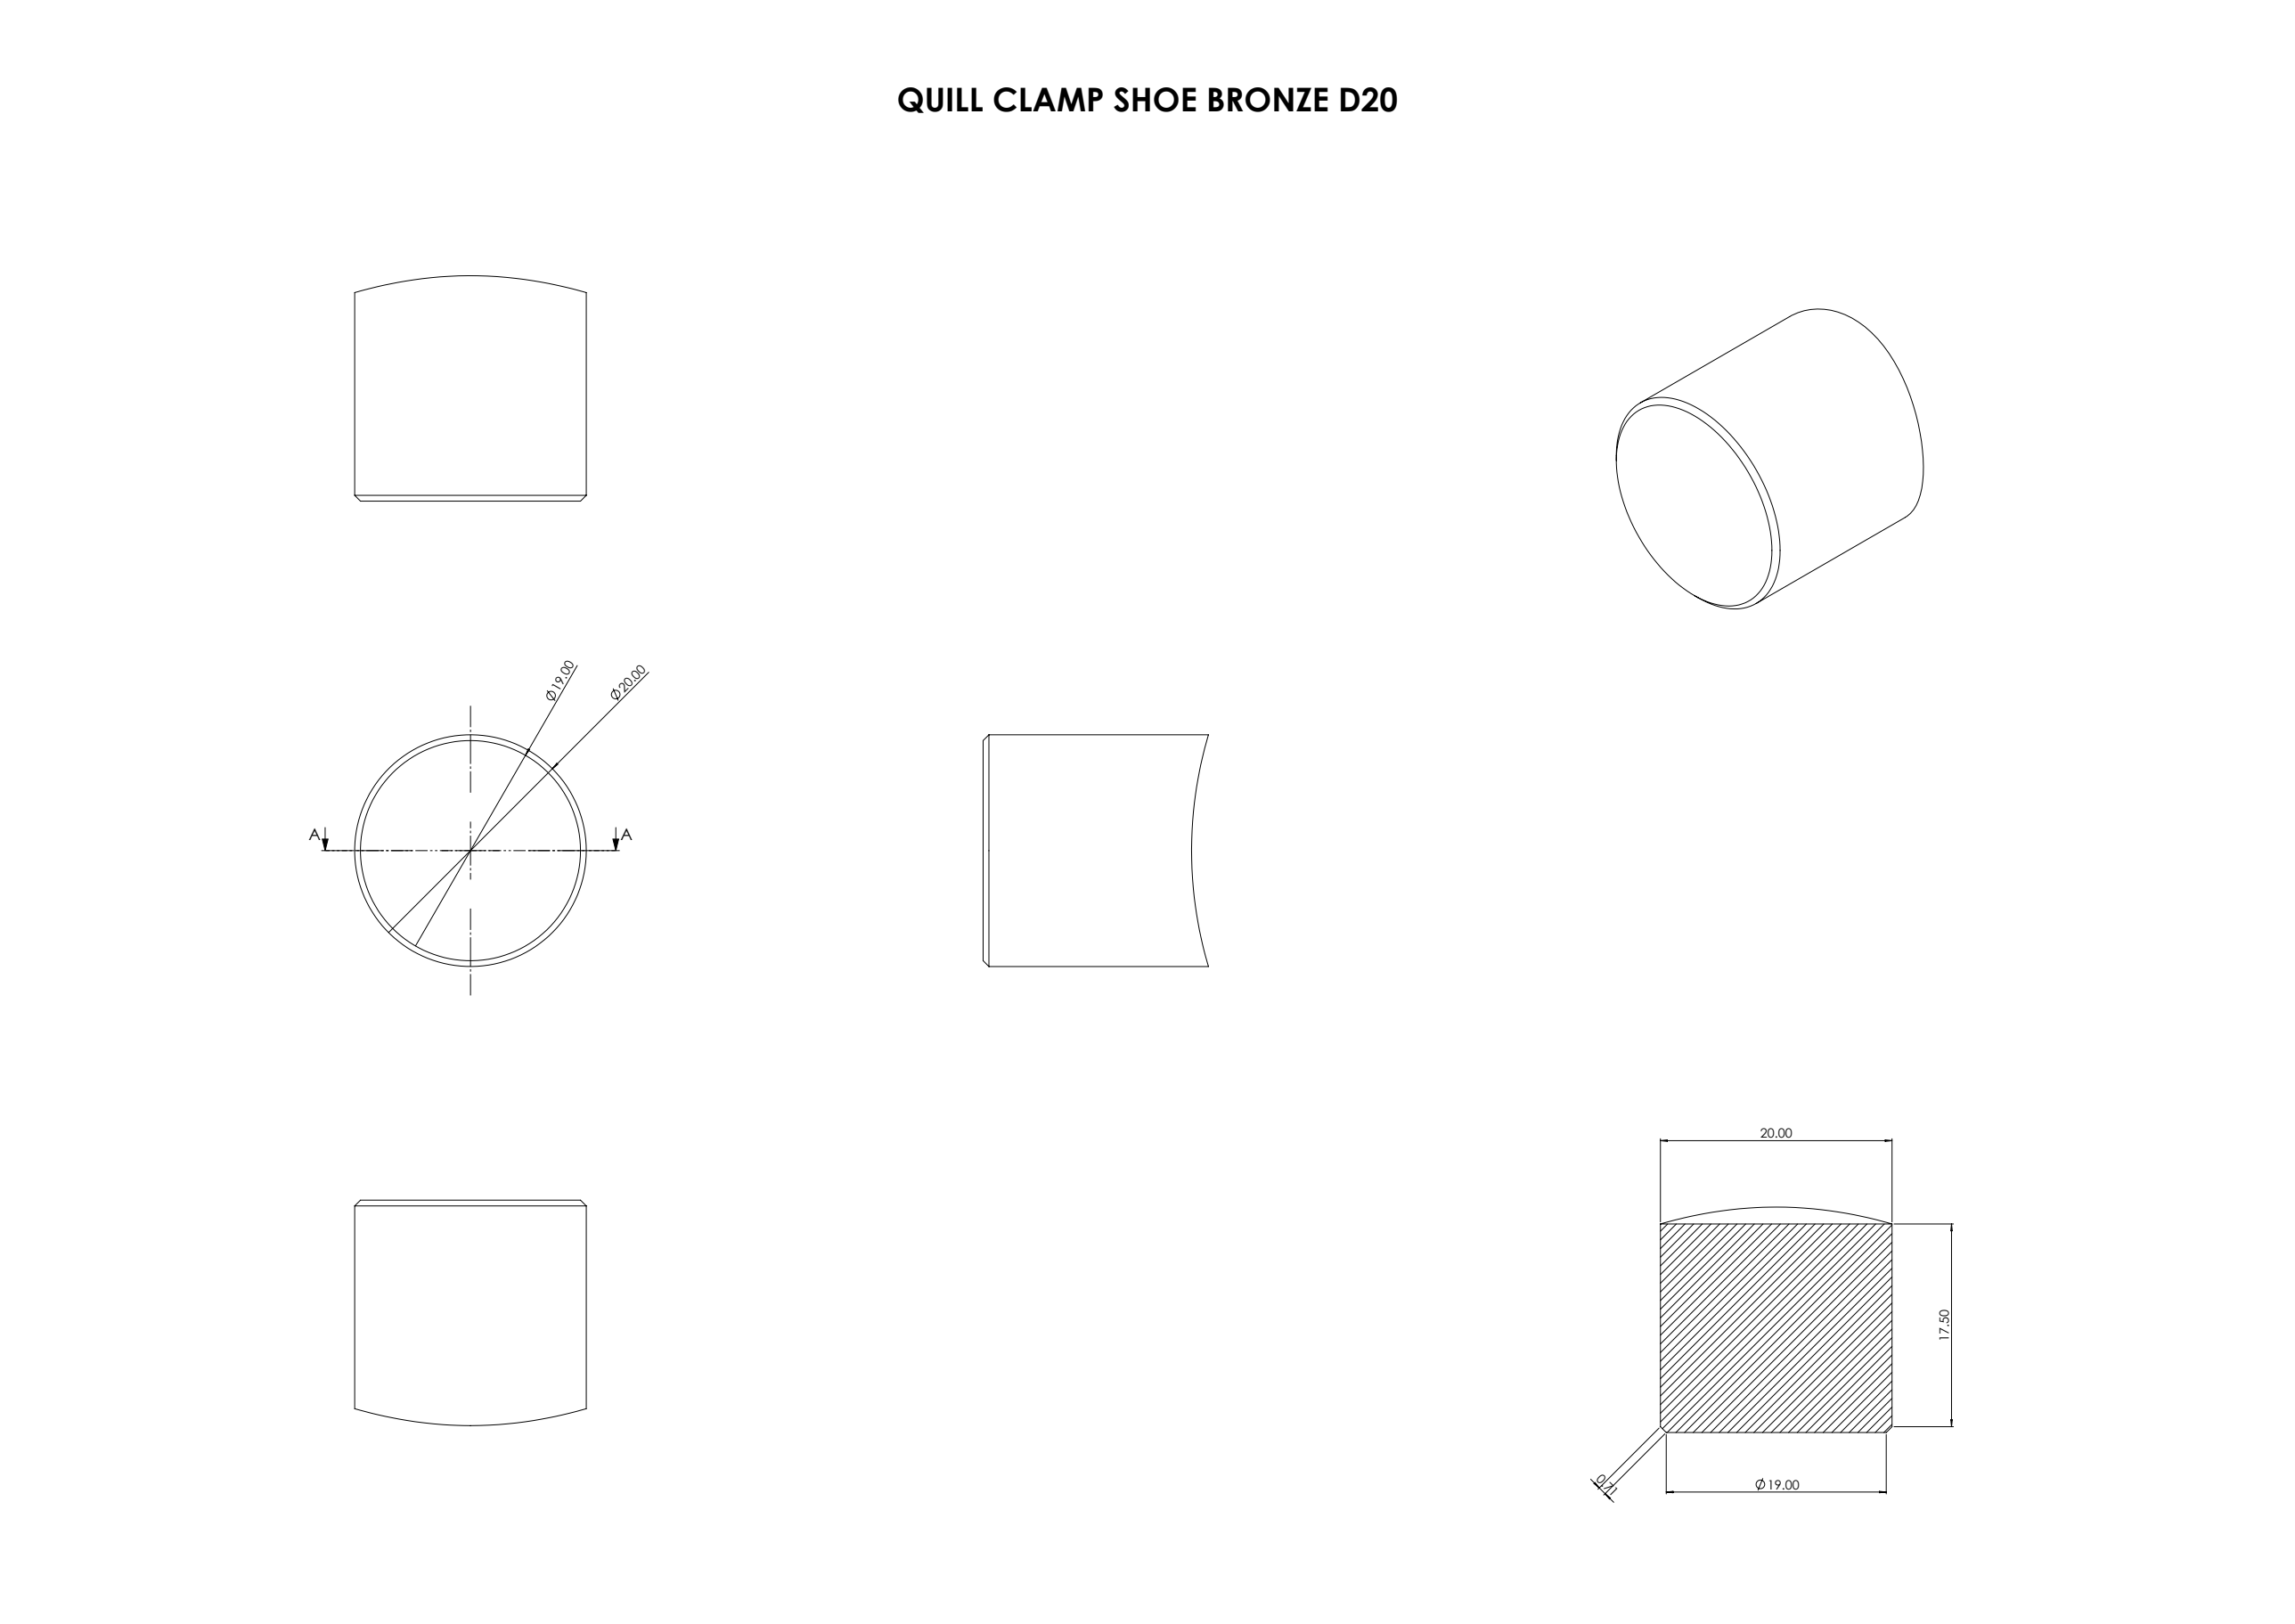
ISO-10303-21;
HEADER;
/* Generated by software containing ST-Developer
 * from STEP Tools, Inc. (www.steptools.com) 
 */

FILE_DESCRIPTION(
/* description */ (''),
/* implementation_level */ '2;1');

FILE_NAME(
/* name */ '13_Quill_Clamp_Shoe_Bronze_D20.step',
/* time_stamp */ '2026-10-26T03:50:32-07:00',
/* author */ (''),
/* organization */ (''),
/* preprocessor_version */ 'ST-DEVELOPER v20.2',
/* originating_system */ 'Autodesk Translation Framework v15.15.0.0',
/* authorisation */ '');

FILE_SCHEMA (('AUTOMOTIVE_DESIGN { 1 0 10303 214 3 1 1 }'));
ENDSEC;

DATA;
#10=MECHANICAL_DESIGN_GEOMETRIC_PRESENTATION_REPRESENTATION('',(#1050),#76660);
#563=B_SPLINE_CURVE_WITH_KNOTS('',3,(#56042,#56043,#56044,#56045,#56046,
#56047,#56048,#56049,#56050,#56051,#56052,#56053,#56054,#56055,#56056,#56057,
#56058,#56059,#56060,#56061,#56062,#56063,#56064,#56065,#56066,#56067),
 .UNSPECIFIED.,.F.,.F.,(4,2,2,2,2,2,2,2,2,2,2,2,4),(0.,0.379021281688117,
0.758042563376235,1.13697172150512,1.515900879634,1.89483003776288,2.27375919589176,
2.65278047757987,3.03180175926799,3.41082304095611,3.78984432264423,4.16877348077311,
4.54770263890199),.UNSPECIFIED.);
#564=B_SPLINE_CURVE_WITH_KNOTS('',3,(#56068,#56069,#56070,#56071,#56072,
#56073,#56074,#56075,#56076,#56077),.UNSPECIFIED.,.F.,.F.,(4,2,2,2,4),(4.54770263890199,
4.92663179703087,5.30556095515975,5.68458223684787,6.06360351853598),
 .UNSPECIFIED.);
#1010=SHAPE_REPRESENTATION_RELATIONSHIP('SRR','None',#76747,#1030);
#1030=ADVANCED_BREP_SHAPE_REPRESENTATION('',(#1070),#76651);
#1050=STYLED_ITEM('',(#76892),#1070);
#1070=MANIFOLD_SOLID_BREP('Clamp shoe',#26675);
#1326=CYLINDRICAL_SURFACE('',#28283,3.5);
#1327=CYLINDRICAL_SURFACE('',#28284,1.);
#2118=PLANE('',#28288);
#3386=FACE_OUTER_BOUND('',#5023,.T.);
#3387=FACE_OUTER_BOUND('',#5024,.T.);
#3388=FACE_OUTER_BOUND('',#5025,.T.);
#3389=FACE_OUTER_BOUND('',#5026,.T.);
#5023=EDGE_LOOP('',(#21447,#21448));
#5024=EDGE_LOOP('',(#21449,#21450,#21451,#21452,#21453));
#5025=EDGE_LOOP('',(#21454,#21455,#21456,#21457));
#5026=EDGE_LOOP('',(#21458));
#6246=CIRCLE('',#28285,1.);
#6247=CIRCLE('',#28287,0.950000000000003);
#7805=LINE('',#56081,#9961);
#7806=LINE('',#56085,#9962);
#9961=VECTOR('',#33320,1.);
#9962=VECTOR('',#33325,0.975000000000001);
#12234=VERTEX_POINT('',#56040);
#12235=VERTEX_POINT('',#56041);
#12236=VERTEX_POINT('',#56079);
#12237=VERTEX_POINT('',#56083);
#15446=EDGE_CURVE('',#12234,#12235,#563,.T.);
#15447=EDGE_CURVE('',#12235,#12234,#564,.T.);
#15448=EDGE_CURVE('',#12236,#12236,#6246,.T.);
#15449=EDGE_CURVE('',#12236,#12235,#7805,.T.);
#15450=EDGE_CURVE('',#12237,#12237,#6247,.T.);
#15451=EDGE_CURVE('',#12237,#12236,#7806,.T.);
#21447=ORIENTED_EDGE('',*,*,#15446,.F.);
#21448=ORIENTED_EDGE('',*,*,#15447,.F.);
#21449=ORIENTED_EDGE('',*,*,#15448,.F.);
#21450=ORIENTED_EDGE('',*,*,#15449,.T.);
#21451=ORIENTED_EDGE('',*,*,#15447,.T.);
#21452=ORIENTED_EDGE('',*,*,#15446,.T.);
#21453=ORIENTED_EDGE('',*,*,#15449,.F.);
#21454=ORIENTED_EDGE('',*,*,#15450,.F.);
#21455=ORIENTED_EDGE('',*,*,#15451,.T.);
#21456=ORIENTED_EDGE('',*,*,#15448,.T.);
#21457=ORIENTED_EDGE('',*,*,#15451,.F.);
#21458=ORIENTED_EDGE('',*,*,#15450,.T.);
#25067=CONICAL_SURFACE('',#28286,0.975000000000001,0.785398163397413);
#25974=ADVANCED_FACE('',(#3386),#1326,.F.);
#25975=ADVANCED_FACE('',(#3387),#1327,.T.);
#25976=ADVANCED_FACE('',(#3388),#25067,.T.);
#25977=ADVANCED_FACE('',(#3389),#2118,.T.);
#26675=CLOSED_SHELL('',(#25974,#25975,#25976,#25977));
#28282=AXIS2_PLACEMENT_3D('',#56038,#33312,#33313);
#28283=AXIS2_PLACEMENT_3D('',#56039,#33314,#33315);
#28284=AXIS2_PLACEMENT_3D('',#56078,#33316,#33317);
#28285=AXIS2_PLACEMENT_3D('',#56080,#33318,#33319);
#28286=AXIS2_PLACEMENT_3D('',#56082,#33321,#33322);
#28287=AXIS2_PLACEMENT_3D('',#56084,#33323,#33324);
#28288=AXIS2_PLACEMENT_3D('',#56086,#33326,#33327);
#33312=DIRECTION('axis',(0.,0.,1.));
#33313=DIRECTION('refdir',(1.,0.,0.));
#33314=DIRECTION('center_axis',(1.,0.,0.));
#33315=DIRECTION('ref_axis',(0.,1.,0.));
#33316=DIRECTION('center_axis',(0.,0.,1.));
#33317=DIRECTION('ref_axis',(1.,0.,0.));
#33318=DIRECTION('center_axis',(0.,0.,1.));
#33319=DIRECTION('ref_axis',(1.,0.,0.));
#33320=DIRECTION('',(0.,0.,-1.));
#33321=DIRECTION('center_axis',(0.,0.,-1.));
#33322=DIRECTION('ref_axis',(1.,0.,0.));
#33323=DIRECTION('center_axis',(0.,0.,1.));
#33324=DIRECTION('ref_axis',(1.,0.,0.));
#33325=DIRECTION('',(-0.707106781186522,-8.65956056235463E-17,-0.707106781186573));
#33326=DIRECTION('center_axis',(0.,0.,1.));
#33327=DIRECTION('ref_axis',(1.,0.,0.));
#56038=CARTESIAN_POINT('',(0.,0.,0.));
#56039=CARTESIAN_POINT('Origin',(33.5,0.,26.5));
#56040=CARTESIAN_POINT('',(33.5,-1.,29.8541019662497));
#56041=CARTESIAN_POINT('',(32.5,-1.16743491188625E-16,30.));
#56042=CARTESIAN_POINT('Ctrl Pts',(33.5,-1.,29.8541019662497));
#56043=CARTESIAN_POINT('Ctrl Pts',(33.6263404272294,-1.,29.8541019662497));
#56044=CARTESIAN_POINT('Ctrl Pts',(33.7605855308726,-0.974606077798943,
29.861986486613));
#56045=CARTESIAN_POINT('Ctrl Pts',(34.006735263926,-0.872342432005776,29.8899599884511));
#56046=CARTESIAN_POINT('Ctrl Pts',(34.1187060914405,-0.795507470932603,
29.9095916302829));
#56047=CARTESIAN_POINT('Ctrl Pts',(34.2954859845766,-0.618727577796462,
29.9460585378213));
#56048=CARTESIAN_POINT('Ctrl Pts',(34.3723376201997,-0.506747952410379,
29.9653343432958));
#56049=CARTESIAN_POINT('Ctrl Pts',(34.4746135319146,-0.260566482292827,
29.9924834581629));
#56050=CARTESIAN_POINT('Ctrl Pts',(34.5,-0.126309719376294,30.));
#56051=CARTESIAN_POINT('Ctrl Pts',(34.5,0.126309719376294,30.));
#56052=CARTESIAN_POINT('Ctrl Pts',(34.4746135319146,0.260566482292828,29.9924834581629));
#56053=CARTESIAN_POINT('Ctrl Pts',(34.3723376201997,0.50674795241038,29.9653343432958));
#56054=CARTESIAN_POINT('Ctrl Pts',(34.2954859845766,0.618727577796462,29.9460585378213));
#56055=CARTESIAN_POINT('Ctrl Pts',(34.1187060914405,0.795507470932603,29.9095916302829));
#56056=CARTESIAN_POINT('Ctrl Pts',(34.006735263926,0.872342432005776,29.8899599884511));
#56057=CARTESIAN_POINT('Ctrl Pts',(33.7605855308726,0.974606077798943,29.861986486613));
#56058=CARTESIAN_POINT('Ctrl Pts',(33.6263404272294,1.,29.8541019662497));
#56059=CARTESIAN_POINT('Ctrl Pts',(33.3736595727706,1.,29.8541019662497));
#56060=CARTESIAN_POINT('Ctrl Pts',(33.2394144691274,0.974606077798943,29.861986486613));
#56061=CARTESIAN_POINT('Ctrl Pts',(32.993264736074,0.872342432005776,29.8899599884511));
#56062=CARTESIAN_POINT('Ctrl Pts',(32.8812939085595,0.795507470932603,29.9095916302829));
#56063=CARTESIAN_POINT('Ctrl Pts',(32.7045140154234,0.618727577796462,29.9460585378213));
#56064=CARTESIAN_POINT('Ctrl Pts',(32.6276623798003,0.506747952410379,29.9653343432958));
#56065=CARTESIAN_POINT('Ctrl Pts',(32.5253864680854,0.260566482292827,29.9924834581629));
#56066=CARTESIAN_POINT('Ctrl Pts',(32.5,0.126309719376294,30.));
#56067=CARTESIAN_POINT('Ctrl Pts',(32.5,3.05311331771918E-16,30.));
#56068=CARTESIAN_POINT('Ctrl Pts',(32.5,-5.55111512312578E-17,30.));
#56069=CARTESIAN_POINT('Ctrl Pts',(32.5,-0.126309719376293,30.));
#56070=CARTESIAN_POINT('Ctrl Pts',(32.5253864680854,-0.260566482292827,
29.9924834581629));
#56071=CARTESIAN_POINT('Ctrl Pts',(32.6276623798003,-0.506747952410379,
29.9653343432958));
#56072=CARTESIAN_POINT('Ctrl Pts',(32.7045140154234,-0.618727577796462,
29.9460585378213));
#56073=CARTESIAN_POINT('Ctrl Pts',(32.8812939085595,-0.795507470932602,
29.9095916302829));
#56074=CARTESIAN_POINT('Ctrl Pts',(32.993264736074,-0.872342432005776,29.8899599884511));
#56075=CARTESIAN_POINT('Ctrl Pts',(33.2394144691274,-0.974606077798943,
29.861986486613));
#56076=CARTESIAN_POINT('Ctrl Pts',(33.3736595727706,-1.,29.8541019662497));
#56077=CARTESIAN_POINT('Ctrl Pts',(33.5,-1.,29.8541019662497));
#56078=CARTESIAN_POINT('Origin',(33.5,0.,30.675));
#56079=CARTESIAN_POINT('',(32.5,-1.22464679914735E-16,31.75));
#56080=CARTESIAN_POINT('Origin',(33.5,0.,31.75));
#56081=CARTESIAN_POINT('',(32.5,-1.22464679914735E-16,30.675));
#56082=CARTESIAN_POINT('Origin',(33.5,0.,31.775));
#56083=CARTESIAN_POINT('',(32.55,-1.16341445918999E-16,31.8));
#56084=CARTESIAN_POINT('Origin',(33.5,0.,31.8));
#56085=CARTESIAN_POINT('',(32.525,-1.19403062916867E-16,31.775));
#56086=CARTESIAN_POINT('Origin',(33.5,0.,31.8));
#76629=UNCERTAINTY_MEASURE_WITH_UNIT(LENGTH_MEASURE(0.001),#76661,
'DISTANCE_ACCURACY_VALUE',
'Maximum model space distance between geometric entities at asserted c
onnectivities');
#76638=UNCERTAINTY_MEASURE_WITH_UNIT(LENGTH_MEASURE(0.001),#76661,
'DISTANCE_ACCURACY_VALUE',
'Maximum model space distance between geometric entities at asserted c
onnectivities');
#76651=(
GEOMETRIC_REPRESENTATION_CONTEXT(3)
GLOBAL_UNCERTAINTY_ASSIGNED_CONTEXT((#76629))
GLOBAL_UNIT_ASSIGNED_CONTEXT((#76661,#76663,#76664))
REPRESENTATION_CONTEXT('','3D')
);
#76660=(
GEOMETRIC_REPRESENTATION_CONTEXT(3)
GLOBAL_UNCERTAINTY_ASSIGNED_CONTEXT((#76638))
GLOBAL_UNIT_ASSIGNED_CONTEXT((#76661,#76663,#76664))
REPRESENTATION_CONTEXT('','3D')
);
#76661=(
LENGTH_UNIT()
NAMED_UNIT(*)
SI_UNIT(.CENTI.,.METRE.)
);
#76663=(
NAMED_UNIT(*)
PLANE_ANGLE_UNIT()
SI_UNIT($,.RADIAN.)
);
#76664=(
NAMED_UNIT(*)
SI_UNIT($,.STERADIAN.)
SOLID_ANGLE_UNIT()
);
#76677=SHAPE_DEFINITION_REPRESENTATION(#76698,#76747);
#76698=PRODUCT_DEFINITION_SHAPE('',$,#76769);
#76747=SHAPE_REPRESENTATION('',(#28282),#76651);
#76756=PRODUCT_DEFINITION_CONTEXT('part definition',#76821,'design');
#76769=PRODUCT_DEFINITION('2026-10-26-11-13-25-360',
'13_Quill_Clamp_Shoe_Bronze_D20',#76790,#76756);
#76790=PRODUCT_DEFINITION_FORMATION('',$,#76835);
#76821=APPLICATION_CONTEXT(
'Core Data for Automotive Mechanical Design Process');
#76822=PRODUCT_CONTEXT('part definition',#76821,'mechanical');
#76835=PRODUCT('2026-10-26-11-13-25-360',
'13_Quill_Clamp_Shoe_Bronze_D20',$,(#76822));
#76886=COLOUR_RGB('Light Blue',0.38,0.62,0.78);
#76887=FILL_AREA_STYLE_COLOUR('',#76886);
#76888=FILL_AREA_STYLE('',(#76887));
#76889=SURFACE_STYLE_FILL_AREA(#76888);
#76890=SURFACE_SIDE_STYLE('',(#76889));
#76891=SURFACE_STYLE_USAGE(.BOTH.,#76890);
#76892=PRESENTATION_STYLE_ASSIGNMENT((#76891));
ENDSEC;
END-ISO-10303-21;
